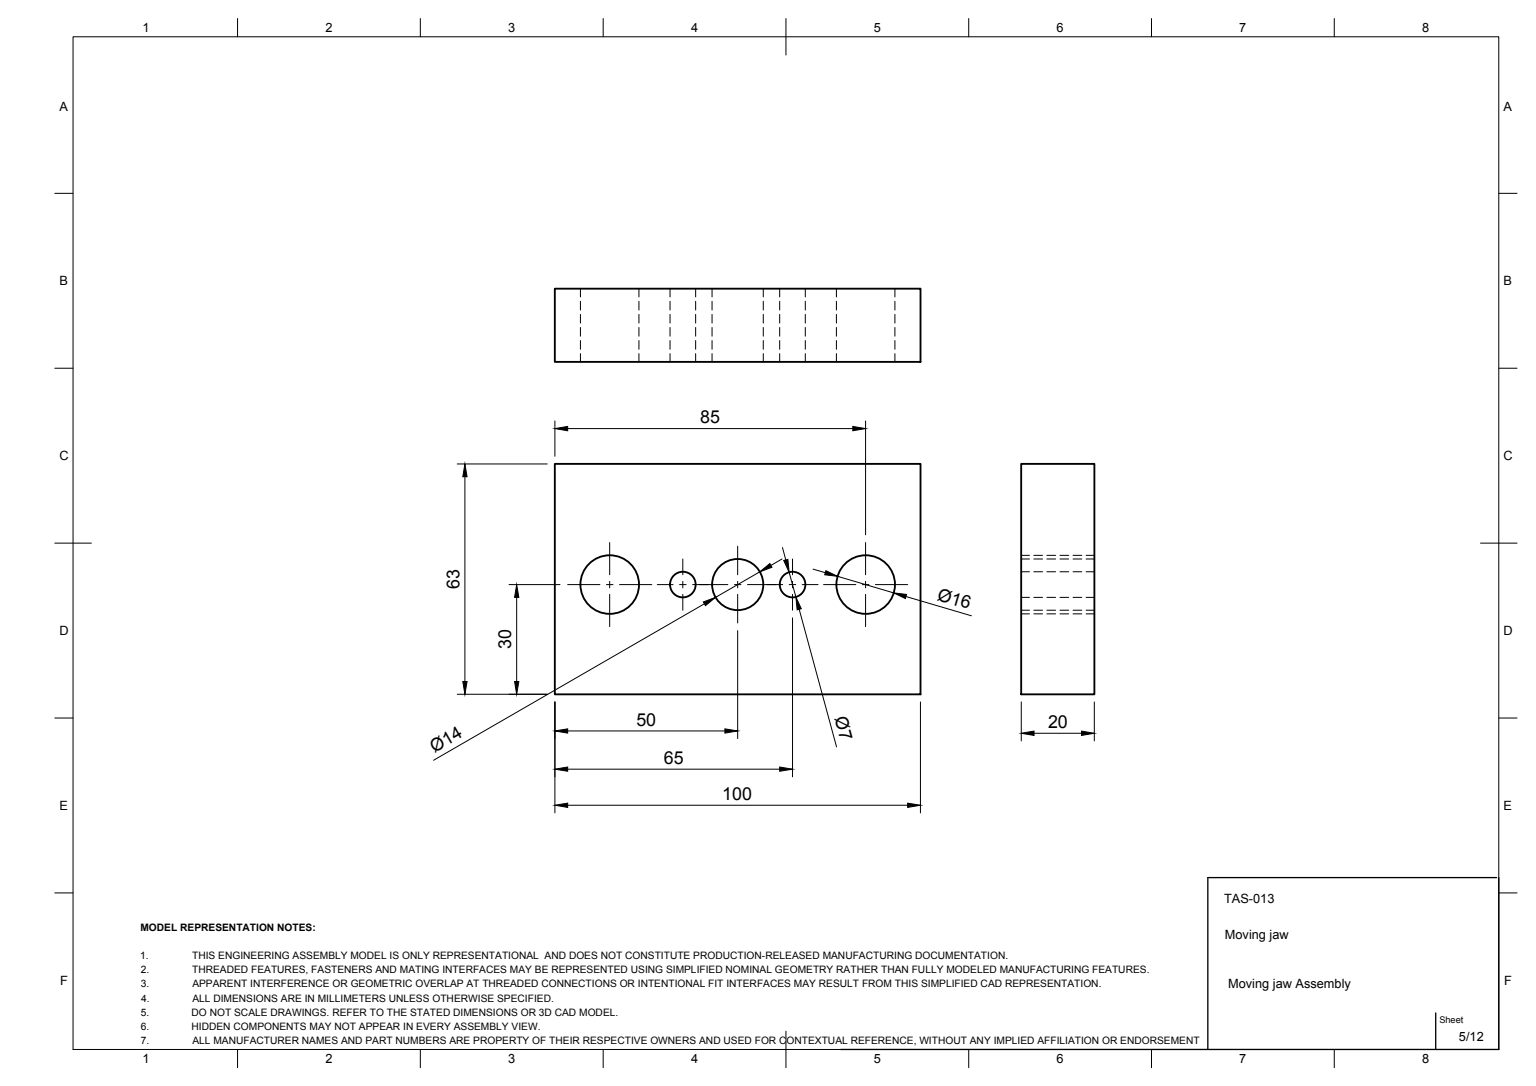
ISO-10303-21;
HEADER;
/* Generated by software containing ST-Developer
 * from STEP Tools, Inc. (www.steptools.com) 
 */

FILE_DESCRIPTION(
/* description */ (
'Independent guided parallel-jaw bracket clamp. Two12mm guide rods, re
placeable bronze sleeves, captured swiveling spindle, replaceable jaw 
pads and modeled M16x2 screw. Native slider/revolute joints linked2mm 
per revolution. Nominal opening0..122 with initial28mm. Base and two i
dentical supports welded. Standard fits, weld details and clamp load r
equire engineering selection.'),
/* implementation_level */ '2;1');

FILE_NAME(
/* name */ 'Moving jaw.step',
/* time_stamp */ '2026-11-14T09:15:44-08:00',
/* author */ (''),
/* organization */ (''),
/* preprocessor_version */ 'ST-DEVELOPER v20.2',
/* originating_system */ 'Autodesk Translation Framework v15.17.0.0',
/* authorisation */ '');

FILE_SCHEMA (('AUTOMOTIVE_DESIGN { 1 0 10303 214 3 1 1 }'));
ENDSEC;

DATA;
#10=MECHANICAL_DESIGN_GEOMETRIC_PRESENTATION_REPRESENTATION('',(#916),#105806);
#892=SHAPE_REPRESENTATION_RELATIONSHIP('SRR','None',#105860,#904);
#904=ADVANCED_BREP_SHAPE_REPRESENTATION('',(#928),#105795);
#916=STYLED_ITEM('',(#105929),#928);
#928=MANIFOLD_SOLID_BREP('Body1',#7203);
#947=FACE_BOUND('',#1365,.T.);
#948=FACE_BOUND('',#1366,.T.);
#949=FACE_BOUND('',#1367,.T.);
#950=FACE_BOUND('',#1368,.T.);
#951=FACE_BOUND('',#1369,.T.);
#952=FACE_BOUND('',#1371,.T.);
#953=FACE_BOUND('',#1372,.T.);
#954=FACE_BOUND('',#1373,.T.);
#955=FACE_BOUND('',#1374,.T.);
#956=FACE_BOUND('',#1375,.T.);
#1004=PLANE('',#7383);
#1005=PLANE('',#7384);
#1006=PLANE('',#7385);
#1007=PLANE('',#7386);
#1008=PLANE('',#7387);
#1009=PLANE('',#7388);
#1075=FACE_OUTER_BOUND('',#1355,.T.);
#1076=FACE_OUTER_BOUND('',#1356,.T.);
#1077=FACE_OUTER_BOUND('',#1357,.T.);
#1078=FACE_OUTER_BOUND('',#1358,.T.);
#1079=FACE_OUTER_BOUND('',#1359,.T.);
#1080=FACE_OUTER_BOUND('',#1360,.T.);
#1081=FACE_OUTER_BOUND('',#1361,.T.);
#1082=FACE_OUTER_BOUND('',#1362,.T.);
#1083=FACE_OUTER_BOUND('',#1363,.T.);
#1084=FACE_OUTER_BOUND('',#1364,.T.);
#1085=FACE_OUTER_BOUND('',#1370,.T.);
#1355=EDGE_LOOP('',(#4461,#4462,#4463,#4464));
#1356=EDGE_LOOP('',(#4465,#4466,#4467,#4468));
#1357=EDGE_LOOP('',(#4469,#4470,#4471,#4472));
#1358=EDGE_LOOP('',(#4473,#4474,#4475,#4476));
#1359=EDGE_LOOP('',(#4477,#4478,#4479,#4480));
#1360=EDGE_LOOP('',(#4481,#4482,#4483,#4484));
#1361=EDGE_LOOP('',(#4485,#4486,#4487,#4488));
#1362=EDGE_LOOP('',(#4489,#4490,#4491,#4492));
#1363=EDGE_LOOP('',(#4493,#4494,#4495,#4496));
#1364=EDGE_LOOP('',(#4497,#4498,#4499,#4500));
#1365=EDGE_LOOP('',(#4501));
#1366=EDGE_LOOP('',(#4502));
#1367=EDGE_LOOP('',(#4503));
#1368=EDGE_LOOP('',(#4504));
#1369=EDGE_LOOP('',(#4505));
#1370=EDGE_LOOP('',(#4506,#4507,#4508,#4509));
#1371=EDGE_LOOP('',(#4510));
#1372=EDGE_LOOP('',(#4511));
#1373=EDGE_LOOP('',(#4512));
#1374=EDGE_LOOP('',(#4513));
#1375=EDGE_LOOP('',(#4514));
#1684=LINE('',#8872,#1964);
#1685=LINE('',#8878,#1965);
#1686=LINE('',#8884,#1966);
#1687=LINE('',#8890,#1967);
#1688=LINE('',#8896,#1968);
#1689=LINE('',#8901,#1969);
#1690=LINE('',#8903,#1970);
#1691=LINE('',#8905,#1971);
#1692=LINE('',#8906,#1972);
#1693=LINE('',#8909,#1973);
#1694=LINE('',#8911,#1974);
#1695=LINE('',#8912,#1975);
#1696=LINE('',#8915,#1976);
#1697=LINE('',#8917,#1977);
#1698=LINE('',#8918,#1978);
#1699=LINE('',#8920,#1979);
#1700=LINE('',#8921,#1980);
#1964=VECTOR('',#7805,3.5);
#1965=VECTOR('',#7812,3.5);
#1966=VECTOR('',#7819,7.);
#1967=VECTOR('',#7826,8.);
#1968=VECTOR('',#7833,8.);
#1969=VECTOR('',#7838,10.);
#1970=VECTOR('',#7839,10.);
#1971=VECTOR('',#7840,10.);
#1972=VECTOR('',#7841,10.);
#1973=VECTOR('',#7844,10.);
#1974=VECTOR('',#7845,10.);
#1975=VECTOR('',#7846,10.);
#1976=VECTOR('',#7849,10.);
#1977=VECTOR('',#7850,10.);
#1978=VECTOR('',#7851,10.);
#1979=VECTOR('',#7854,10.);
#1980=VECTOR('',#7855,10.);
#2236=CIRCLE('',#7369,3.5);
#2237=CIRCLE('',#7370,3.5);
#2238=CIRCLE('',#7372,3.5);
#2239=CIRCLE('',#7373,3.5);
#2240=CIRCLE('',#7375,7.);
#2241=CIRCLE('',#7376,7.);
#2242=CIRCLE('',#7378,8.);
#2243=CIRCLE('',#7379,8.);
#2244=CIRCLE('',#7381,8.);
#2245=CIRCLE('',#7382,8.);
#2342=VERTEX_POINT('',#8869);
#2343=VERTEX_POINT('',#8871);
#2344=VERTEX_POINT('',#8875);
#2345=VERTEX_POINT('',#8877);
#2346=VERTEX_POINT('',#8881);
#2347=VERTEX_POINT('',#8883);
#2348=VERTEX_POINT('',#8887);
#2349=VERTEX_POINT('',#8889);
#2350=VERTEX_POINT('',#8893);
#2351=VERTEX_POINT('',#8895);
#2352=VERTEX_POINT('',#8899);
#2353=VERTEX_POINT('',#8900);
#2354=VERTEX_POINT('',#8902);
#2355=VERTEX_POINT('',#8904);
#2356=VERTEX_POINT('',#8908);
#2357=VERTEX_POINT('',#8910);
#2358=VERTEX_POINT('',#8914);
#2359=VERTEX_POINT('',#8916);
#3275=EDGE_CURVE('',#2342,#2342,#2236,.T.);
#3276=EDGE_CURVE('',#2342,#2343,#1684,.T.);
#3277=EDGE_CURVE('',#2343,#2343,#2237,.T.);
#3278=EDGE_CURVE('',#2344,#2344,#2238,.T.);
#3279=EDGE_CURVE('',#2344,#2345,#1685,.T.);
#3280=EDGE_CURVE('',#2345,#2345,#2239,.T.);
#3281=EDGE_CURVE('',#2346,#2346,#2240,.T.);
#3282=EDGE_CURVE('',#2346,#2347,#1686,.T.);
#3283=EDGE_CURVE('',#2347,#2347,#2241,.T.);
#3284=EDGE_CURVE('',#2348,#2348,#2242,.T.);
#3285=EDGE_CURVE('',#2348,#2349,#1687,.T.);
#3286=EDGE_CURVE('',#2349,#2349,#2243,.T.);
#3287=EDGE_CURVE('',#2350,#2350,#2244,.T.);
#3288=EDGE_CURVE('',#2350,#2351,#1688,.T.);
#3289=EDGE_CURVE('',#2351,#2351,#2245,.T.);
#3290=EDGE_CURVE('',#2352,#2353,#1689,.F.);
#3291=EDGE_CURVE('',#2353,#2354,#1690,.T.);
#3292=EDGE_CURVE('',#2355,#2354,#1691,.F.);
#3293=EDGE_CURVE('',#2352,#2355,#1692,.F.);
#3294=EDGE_CURVE('',#2356,#2352,#1693,.T.);
#3295=EDGE_CURVE('',#2357,#2355,#1694,.T.);
#3296=EDGE_CURVE('',#2356,#2357,#1695,.T.);
#3297=EDGE_CURVE('',#2358,#2356,#1696,.T.);
#3298=EDGE_CURVE('',#2359,#2357,#1697,.T.);
#3299=EDGE_CURVE('',#2358,#2359,#1698,.T.);
#3300=EDGE_CURVE('',#2353,#2358,#1699,.T.);
#3301=EDGE_CURVE('',#2354,#2359,#1700,.T.);
#4461=ORIENTED_EDGE('',*,*,#3275,.F.);
#4462=ORIENTED_EDGE('',*,*,#3276,.T.);
#4463=ORIENTED_EDGE('',*,*,#3277,.F.);
#4464=ORIENTED_EDGE('',*,*,#3276,.F.);
#4465=ORIENTED_EDGE('',*,*,#3278,.F.);
#4466=ORIENTED_EDGE('',*,*,#3279,.T.);
#4467=ORIENTED_EDGE('',*,*,#3280,.F.);
#4468=ORIENTED_EDGE('',*,*,#3279,.F.);
#4469=ORIENTED_EDGE('',*,*,#3281,.F.);
#4470=ORIENTED_EDGE('',*,*,#3282,.T.);
#4471=ORIENTED_EDGE('',*,*,#3283,.F.);
#4472=ORIENTED_EDGE('',*,*,#3282,.F.);
#4473=ORIENTED_EDGE('',*,*,#3284,.F.);
#4474=ORIENTED_EDGE('',*,*,#3285,.T.);
#4475=ORIENTED_EDGE('',*,*,#3286,.F.);
#4476=ORIENTED_EDGE('',*,*,#3285,.F.);
#4477=ORIENTED_EDGE('',*,*,#3287,.F.);
#4478=ORIENTED_EDGE('',*,*,#3288,.T.);
#4479=ORIENTED_EDGE('',*,*,#3289,.F.);
#4480=ORIENTED_EDGE('',*,*,#3288,.F.);
#4481=ORIENTED_EDGE('',*,*,#3290,.T.);
#4482=ORIENTED_EDGE('',*,*,#3291,.T.);
#4483=ORIENTED_EDGE('',*,*,#3292,.F.);
#4484=ORIENTED_EDGE('',*,*,#3293,.F.);
#4485=ORIENTED_EDGE('',*,*,#3294,.T.);
#4486=ORIENTED_EDGE('',*,*,#3293,.T.);
#4487=ORIENTED_EDGE('',*,*,#3295,.F.);
#4488=ORIENTED_EDGE('',*,*,#3296,.F.);
#4489=ORIENTED_EDGE('',*,*,#3297,.T.);
#4490=ORIENTED_EDGE('',*,*,#3296,.T.);
#4491=ORIENTED_EDGE('',*,*,#3298,.F.);
#4492=ORIENTED_EDGE('',*,*,#3299,.F.);
#4493=ORIENTED_EDGE('',*,*,#3300,.T.);
#4494=ORIENTED_EDGE('',*,*,#3299,.T.);
#4495=ORIENTED_EDGE('',*,*,#3301,.F.);
#4496=ORIENTED_EDGE('',*,*,#3291,.F.);
#4497=ORIENTED_EDGE('',*,*,#3301,.T.);
#4498=ORIENTED_EDGE('',*,*,#3298,.T.);
#4499=ORIENTED_EDGE('',*,*,#3295,.T.);
#4500=ORIENTED_EDGE('',*,*,#3292,.T.);
#4501=ORIENTED_EDGE('',*,*,#3275,.T.);
#4502=ORIENTED_EDGE('',*,*,#3278,.T.);
#4503=ORIENTED_EDGE('',*,*,#3281,.T.);
#4504=ORIENTED_EDGE('',*,*,#3284,.T.);
#4505=ORIENTED_EDGE('',*,*,#3287,.T.);
#4506=ORIENTED_EDGE('',*,*,#3300,.F.);
#4507=ORIENTED_EDGE('',*,*,#3290,.F.);
#4508=ORIENTED_EDGE('',*,*,#3294,.F.);
#4509=ORIENTED_EDGE('',*,*,#3297,.F.);
#4510=ORIENTED_EDGE('',*,*,#3277,.T.);
#4511=ORIENTED_EDGE('',*,*,#3280,.T.);
#4512=ORIENTED_EDGE('',*,*,#3283,.T.);
#4513=ORIENTED_EDGE('',*,*,#3286,.T.);
#4514=ORIENTED_EDGE('',*,*,#3289,.T.);
#6741=CYLINDRICAL_SURFACE('',#7368,3.5);
#6742=CYLINDRICAL_SURFACE('',#7371,3.5);
#6743=CYLINDRICAL_SURFACE('',#7374,7.);
#6744=CYLINDRICAL_SURFACE('',#7377,8.);
#6745=CYLINDRICAL_SURFACE('',#7380,8.);
#6940=ADVANCED_FACE('',(#1075),#6741,.F.);
#6941=ADVANCED_FACE('',(#1076),#6742,.F.);
#6942=ADVANCED_FACE('',(#1077),#6743,.F.);
#6943=ADVANCED_FACE('',(#1078),#6744,.F.);
#6944=ADVANCED_FACE('',(#1079),#6745,.F.);
#6945=ADVANCED_FACE('',(#1080),#1004,.T.);
#6946=ADVANCED_FACE('',(#1081),#1005,.T.);
#6947=ADVANCED_FACE('',(#1082),#1006,.T.);
#6948=ADVANCED_FACE('',(#1083),#1007,.T.);
#6949=ADVANCED_FACE('',(#1084,#947,#948,#949,#950,#951),#1008,.T.);
#6950=ADVANCED_FACE('',(#1085,#952,#953,#954,#955,#956),#1009,.F.);
#7203=CLOSED_SHELL('',(#6940,#6941,#6942,#6943,#6944,#6945,#6946,#6947,
#6948,#6949,#6950));
#7367=AXIS2_PLACEMENT_3D('',#8867,#7799,#7800);
#7368=AXIS2_PLACEMENT_3D('',#8868,#7801,#7802);
#7369=AXIS2_PLACEMENT_3D('',#8870,#7803,#7804);
#7370=AXIS2_PLACEMENT_3D('',#8873,#7806,#7807);
#7371=AXIS2_PLACEMENT_3D('',#8874,#7808,#7809);
#7372=AXIS2_PLACEMENT_3D('',#8876,#7810,#7811);
#7373=AXIS2_PLACEMENT_3D('',#8879,#7813,#7814);
#7374=AXIS2_PLACEMENT_3D('',#8880,#7815,#7816);
#7375=AXIS2_PLACEMENT_3D('',#8882,#7817,#7818);
#7376=AXIS2_PLACEMENT_3D('',#8885,#7820,#7821);
#7377=AXIS2_PLACEMENT_3D('',#8886,#7822,#7823);
#7378=AXIS2_PLACEMENT_3D('',#8888,#7824,#7825);
#7379=AXIS2_PLACEMENT_3D('',#8891,#7827,#7828);
#7380=AXIS2_PLACEMENT_3D('',#8892,#7829,#7830);
#7381=AXIS2_PLACEMENT_3D('',#8894,#7831,#7832);
#7382=AXIS2_PLACEMENT_3D('',#8897,#7834,#7835);
#7383=AXIS2_PLACEMENT_3D('',#8898,#7836,#7837);
#7384=AXIS2_PLACEMENT_3D('',#8907,#7842,#7843);
#7385=AXIS2_PLACEMENT_3D('',#8913,#7847,#7848);
#7386=AXIS2_PLACEMENT_3D('',#8919,#7852,#7853);
#7387=AXIS2_PLACEMENT_3D('',#8922,#7856,#7857);
#7388=AXIS2_PLACEMENT_3D('',#8923,#7858,#7859);
#7799=DIRECTION('axis',(0.,0.,1.));
#7800=DIRECTION('refdir',(1.,0.,0.));
#7801=DIRECTION('center_axis',(0.,0.,-1.));
#7802=DIRECTION('ref_axis',(1.,0.,0.));
#7803=DIRECTION('center_axis',(0.,0.,-1.));
#7804=DIRECTION('ref_axis',(1.,0.,0.));
#7805=DIRECTION('',(0.,0.,-1.));
#7806=DIRECTION('center_axis',(0.,0.,1.));
#7807=DIRECTION('ref_axis',(1.,0.,0.));
#7808=DIRECTION('center_axis',(0.,0.,-1.));
#7809=DIRECTION('ref_axis',(1.,0.,0.));
#7810=DIRECTION('center_axis',(0.,0.,-1.));
#7811=DIRECTION('ref_axis',(1.,0.,0.));
#7812=DIRECTION('',(0.,0.,-1.));
#7813=DIRECTION('center_axis',(0.,0.,1.));
#7814=DIRECTION('ref_axis',(1.,0.,0.));
#7815=DIRECTION('center_axis',(0.,0.,-1.));
#7816=DIRECTION('ref_axis',(1.,0.,0.));
#7817=DIRECTION('center_axis',(0.,0.,-1.));
#7818=DIRECTION('ref_axis',(1.,0.,0.));
#7819=DIRECTION('',(0.,0.,-1.));
#7820=DIRECTION('center_axis',(0.,0.,1.));
#7821=DIRECTION('ref_axis',(1.,0.,0.));
#7822=DIRECTION('center_axis',(0.,0.,-1.));
#7823=DIRECTION('ref_axis',(1.,0.,0.));
#7824=DIRECTION('center_axis',(0.,0.,-1.));
#7825=DIRECTION('ref_axis',(1.,0.,0.));
#7826=DIRECTION('',(0.,0.,-1.));
#7827=DIRECTION('center_axis',(0.,0.,1.));
#7828=DIRECTION('ref_axis',(1.,0.,0.));
#7829=DIRECTION('center_axis',(0.,0.,-1.));
#7830=DIRECTION('ref_axis',(1.,0.,0.));
#7831=DIRECTION('center_axis',(0.,0.,-1.));
#7832=DIRECTION('ref_axis',(1.,0.,0.));
#7833=DIRECTION('',(0.,0.,-1.));
#7834=DIRECTION('center_axis',(0.,0.,1.));
#7835=DIRECTION('ref_axis',(1.,0.,0.));
#7836=DIRECTION('center_axis',(0.,1.,0.));
#7837=DIRECTION('ref_axis',(-1.,0.,0.));
#7838=DIRECTION('',(1.,0.,0.));
#7839=DIRECTION('',(0.,0.,1.));
#7840=DIRECTION('',(1.,0.,0.));
#7841=DIRECTION('',(0.,0.,-1.));
#7842=DIRECTION('center_axis',(1.,0.,0.));
#7843=DIRECTION('ref_axis',(0.,1.,0.));
#7844=DIRECTION('',(0.,1.,0.));
#7845=DIRECTION('',(0.,1.,0.));
#7846=DIRECTION('',(0.,0.,1.));
#7847=DIRECTION('center_axis',(0.,-1.,0.));
#7848=DIRECTION('ref_axis',(1.,0.,0.));
#7849=DIRECTION('',(1.,0.,0.));
#7850=DIRECTION('',(1.,0.,0.));
#7851=DIRECTION('',(0.,0.,1.));
#7852=DIRECTION('center_axis',(-1.,0.,0.));
#7853=DIRECTION('ref_axis',(0.,-1.,0.));
#7854=DIRECTION('',(0.,-1.,0.));
#7855=DIRECTION('',(0.,-1.,0.));
#7856=DIRECTION('center_axis',(0.,0.,1.));
#7857=DIRECTION('ref_axis',(1.,0.,0.));
#7858=DIRECTION('center_axis',(0.,0.,1.));
#7859=DIRECTION('ref_axis',(1.,0.,0.));
#8867=CARTESIAN_POINT('',(0.,0.,0.));
#8868=CARTESIAN_POINT('Origin',(-15.,0.,10.));
#8869=CARTESIAN_POINT('',(-18.5,4.28626379701574E-16,20.));
#8870=CARTESIAN_POINT('Origin',(-15.,0.,20.));
#8871=CARTESIAN_POINT('',(-18.5,4.28626379701574E-16,0.));
#8872=CARTESIAN_POINT('',(-18.5,4.28626379701574E-16,10.));
#8873=CARTESIAN_POINT('Origin',(-15.,0.,0.));
#8874=CARTESIAN_POINT('Origin',(15.,0.,10.));
#8875=CARTESIAN_POINT('',(11.5,4.28626379701574E-16,20.));
#8876=CARTESIAN_POINT('Origin',(15.,0.,20.));
#8877=CARTESIAN_POINT('',(11.5,4.28626379701574E-16,0.));
#8878=CARTESIAN_POINT('',(11.5,4.28626379701574E-16,10.));
#8879=CARTESIAN_POINT('Origin',(15.,0.,0.));
#8880=CARTESIAN_POINT('Origin',(0.,0.,10.));
#8881=CARTESIAN_POINT('',(-7.,8.57252759403147E-16,20.));
#8882=CARTESIAN_POINT('Origin',(0.,0.,20.));
#8883=CARTESIAN_POINT('',(-7.,8.57252759403147E-16,0.));
#8884=CARTESIAN_POINT('',(-7.,8.57252759403147E-16,10.));
#8885=CARTESIAN_POINT('Origin',(0.,0.,0.));
#8886=CARTESIAN_POINT('Origin',(-35.,0.,10.));
#8887=CARTESIAN_POINT('',(-43.,9.79717439317883E-16,20.));
#8888=CARTESIAN_POINT('Origin',(-35.,0.,20.));
#8889=CARTESIAN_POINT('',(-43.,9.79717439317883E-16,0.));
#8890=CARTESIAN_POINT('',(-43.,9.79717439317883E-16,10.));
#8891=CARTESIAN_POINT('Origin',(-35.,0.,0.));
#8892=CARTESIAN_POINT('Origin',(35.,0.,10.));
#8893=CARTESIAN_POINT('',(27.,9.79717439317883E-16,20.));
#8894=CARTESIAN_POINT('Origin',(35.,0.,20.));
#8895=CARTESIAN_POINT('',(27.,9.79717439317883E-16,0.));
#8896=CARTESIAN_POINT('',(27.,9.79717439317883E-16,10.));
#8897=CARTESIAN_POINT('Origin',(35.,0.,0.));
#8898=CARTESIAN_POINT('Origin',(50.,33.,0.));
#8899=CARTESIAN_POINT('',(50.,33.,0.));
#8900=CARTESIAN_POINT('',(-50.,33.,0.));
#8901=CARTESIAN_POINT('',(25.,33.,0.));
#8902=CARTESIAN_POINT('',(-50.,33.,20.));
#8903=CARTESIAN_POINT('',(-50.,33.,0.));
#8904=CARTESIAN_POINT('',(50.,33.,20.));
#8905=CARTESIAN_POINT('',(25.,33.,20.));
#8906=CARTESIAN_POINT('',(50.,33.,0.));
#8907=CARTESIAN_POINT('Origin',(50.,-30.,0.));
#8908=CARTESIAN_POINT('',(50.,-30.,0.));
#8909=CARTESIAN_POINT('',(50.,-30.,0.));
#8910=CARTESIAN_POINT('',(50.,-30.,20.));
#8911=CARTESIAN_POINT('',(50.,-30.,20.));
#8912=CARTESIAN_POINT('',(50.,-30.,0.));
#8913=CARTESIAN_POINT('Origin',(-50.,-30.,0.));
#8914=CARTESIAN_POINT('',(-50.,-30.,0.));
#8915=CARTESIAN_POINT('',(-50.,-30.,0.));
#8916=CARTESIAN_POINT('',(-50.,-30.,20.));
#8917=CARTESIAN_POINT('',(-50.,-30.,20.));
#8918=CARTESIAN_POINT('',(-50.,-30.,0.));
#8919=CARTESIAN_POINT('Origin',(-50.,30.,0.));
#8920=CARTESIAN_POINT('',(-50.,30.,0.));
#8921=CARTESIAN_POINT('',(-50.,30.,20.));
#8922=CARTESIAN_POINT('Origin',(0.,0.,20.));
#8923=CARTESIAN_POINT('Origin',(0.,0.,0.));
#105781=UNCERTAINTY_MEASURE_WITH_UNIT(LENGTH_MEASURE(0.01),#105807,
'DISTANCE_ACCURACY_VALUE',
'Maximum model space distance between geometric entities at asserted c
onnectivities');
#105792=UNCERTAINTY_MEASURE_WITH_UNIT(LENGTH_MEASURE(0.01),#105807,
'DISTANCE_ACCURACY_VALUE',
'Maximum model space distance between geometric entities at asserted c
onnectivities');
#105795=(
GEOMETRIC_REPRESENTATION_CONTEXT(3)
GLOBAL_UNCERTAINTY_ASSIGNED_CONTEXT((#105781))
GLOBAL_UNIT_ASSIGNED_CONTEXT((#105807,#105809,#105810))
REPRESENTATION_CONTEXT('','3D')
);
#105806=(
GEOMETRIC_REPRESENTATION_CONTEXT(3)
GLOBAL_UNCERTAINTY_ASSIGNED_CONTEXT((#105792))
GLOBAL_UNIT_ASSIGNED_CONTEXT((#105807,#105809,#105810))
REPRESENTATION_CONTEXT('','3D')
);
#105807=(
LENGTH_UNIT()
NAMED_UNIT(*)
SI_UNIT(.MILLI.,.METRE.)
);
#105809=(
NAMED_UNIT(*)
PLANE_ANGLE_UNIT()
SI_UNIT($,.RADIAN.)
);
#105810=(
NAMED_UNIT(*)
SI_UNIT($,.STERADIAN.)
SOLID_ANGLE_UNIT()
);
#105813=SHAPE_DEFINITION_REPRESENTATION(#105826,#105860);
#105826=PRODUCT_DEFINITION_SHAPE('',$,#105874);
#105860=SHAPE_REPRESENTATION('',(#7367),#105795);
#105871=PRODUCT_DEFINITION_CONTEXT('part definition',#105912,'design');
#105874=PRODUCT_DEFINITION('Moving jaw','Moving jaw',#105887,#105871);
#105887=PRODUCT_DEFINITION_FORMATION('',$,#105916);
#105912=APPLICATION_CONTEXT(
'Core Data for Automotive Mechanical Design Process');
#105913=PRODUCT_CONTEXT('part definition',#105912,'mechanical');
#105916=PRODUCT('Moving jaw','Moving jaw','Moving jaw',(#105913));
#105929=PRESENTATION_STYLE_ASSIGNMENT((#105935));
#105935=SURFACE_STYLE_USAGE(.BOTH.,#105941);
#105941=SURFACE_SIDE_STYLE('',(#105947));
#105947=SURFACE_STYLE_FILL_AREA(#105953);
#105953=FILL_AREA_STYLE('Opaque(81,175,227)',(#105959));
#105959=FILL_AREA_STYLE_COLOUR('Opaque(81,175,227)',#105965);
#105965=COLOUR_RGB('Opaque(81,175,227)',0.317647058823529,0.686274509803922,
0.890196078431372);
ENDSEC;
END-ISO-10303-21;
